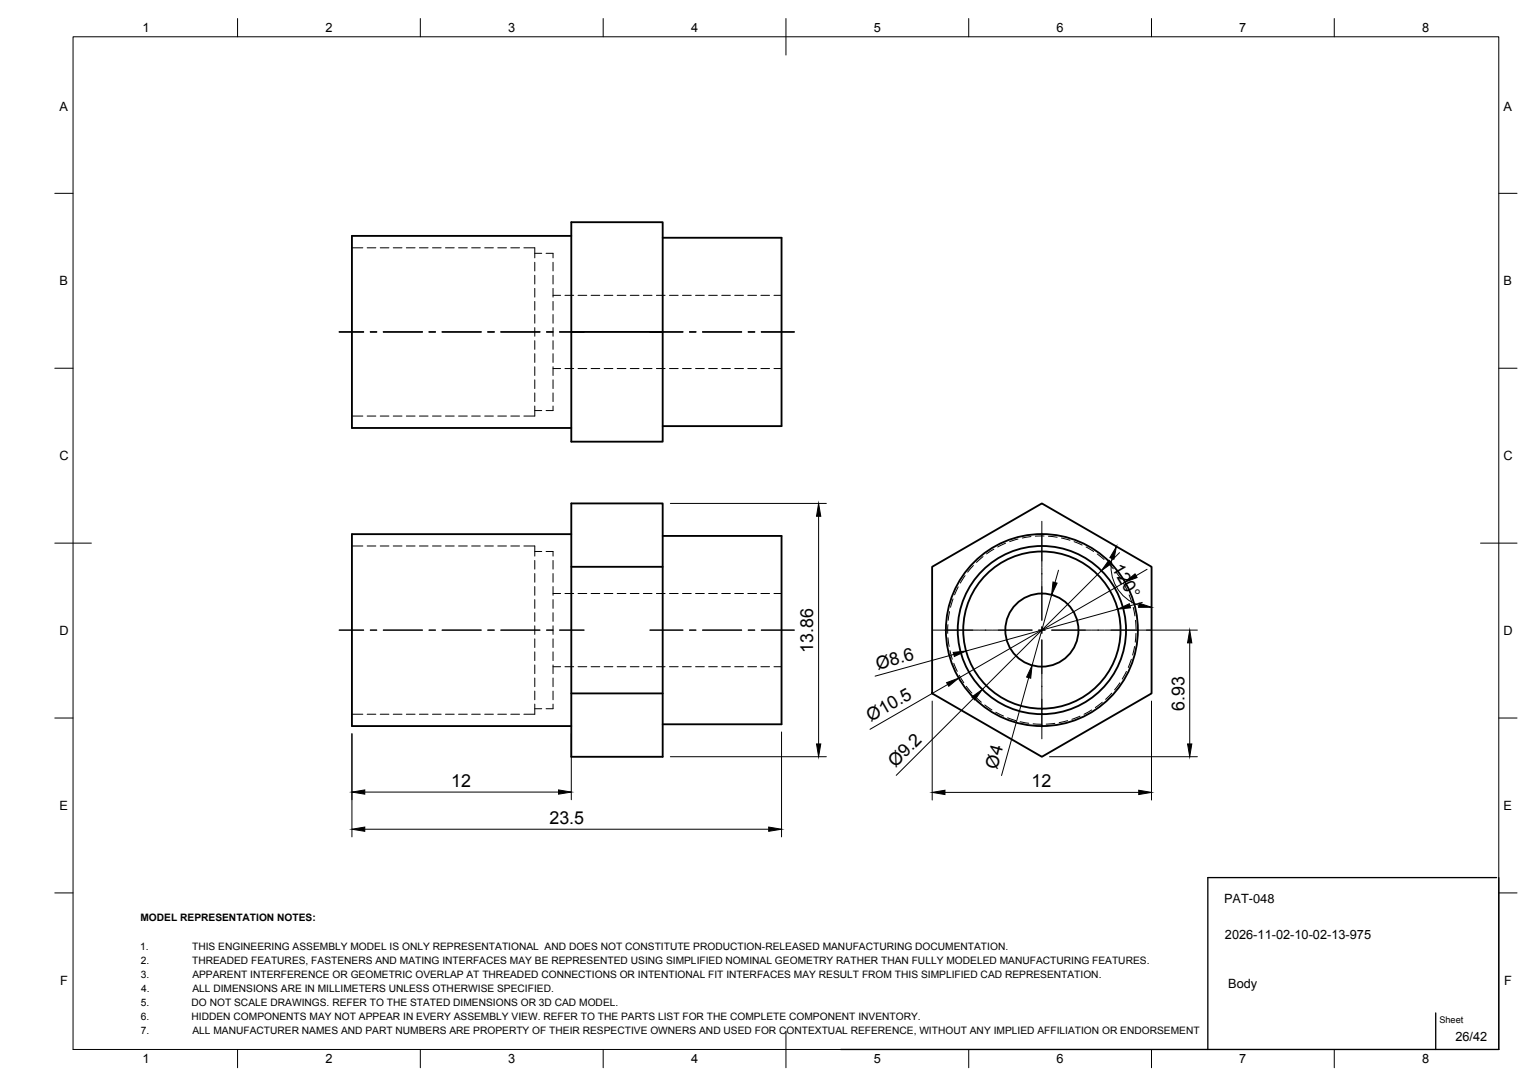
ISO-10303-21;
HEADER;
/* Generated by software containing ST-Developer
 * from STEP Tools, Inc. (www.steptools.com) 
 */

FILE_DESCRIPTION(
/* description */ ('Guided pneumatic stop gate'),
/* implementation_level */ '2;1');

FILE_NAME(
/* name */ 'Body.step',
/* time_stamp */ '2026-10-27T21:43:45-07:00',
/* author */ (''),
/* organization */ (''),
/* preprocessor_version */ 'ST-DEVELOPER v20.2',
/* originating_system */ 'Autodesk Translation Framework v15.17.0.0',
/* authorisation */ '');

FILE_SCHEMA (('AUTOMOTIVE_DESIGN { 1 0 10303 214 3 1 1 }'));
ENDSEC;

DATA;
#10=MECHANICAL_DESIGN_GEOMETRIC_PRESENTATION_REPRESENTATION('',(#546),#14392);
#462=SHAPE_REPRESENTATION_RELATIONSHIP('SRR','None',#14597,#504);
#504=ADVANCED_BREP_SHAPE_REPRESENTATION('',(#587),#14359);
#546=STYLED_ITEM('',(#14870),#587);
#587=MANIFOLD_SOLID_BREP('Body1',#7887);
#682=FACE_BOUND('',#1842,.T.);
#683=FACE_BOUND('',#1844,.T.);
#684=FACE_BOUND('',#1846,.T.);
#685=FACE_BOUND('',#1854,.T.);
#686=FACE_BOUND('',#1857,.T.);
#687=FACE_BOUND('',#1861,.T.);
#948=PLANE('',#8728);
#949=PLANE('',#8730);
#950=PLANE('',#8732);
#951=PLANE('',#8734);
#952=PLANE('',#8735);
#953=PLANE('',#8736);
#954=PLANE('',#8737);
#955=PLANE('',#8738);
#956=PLANE('',#8739);
#957=PLANE('',#8740);
#958=PLANE('',#8744);
#959=PLANE('',#8749);
#1298=FACE_OUTER_BOUND('',#1840,.T.);
#1299=FACE_OUTER_BOUND('',#1841,.T.);
#1300=FACE_OUTER_BOUND('',#1843,.T.);
#1301=FACE_OUTER_BOUND('',#1845,.T.);
#1302=FACE_OUTER_BOUND('',#1847,.T.);
#1303=FACE_OUTER_BOUND('',#1848,.T.);
#1304=FACE_OUTER_BOUND('',#1849,.T.);
#1305=FACE_OUTER_BOUND('',#1850,.T.);
#1306=FACE_OUTER_BOUND('',#1851,.T.);
#1307=FACE_OUTER_BOUND('',#1852,.T.);
#1308=FACE_OUTER_BOUND('',#1853,.T.);
#1309=FACE_OUTER_BOUND('',#1855,.T.);
#1310=FACE_OUTER_BOUND('',#1856,.T.);
#1311=FACE_OUTER_BOUND('',#1858,.T.);
#1312=FACE_OUTER_BOUND('',#1859,.T.);
#1313=FACE_OUTER_BOUND('',#1860,.T.);
#1314=FACE_OUTER_BOUND('',#1862,.T.);
#1840=EDGE_LOOP('',(#6034,#6035,#6036,#6037));
#1841=EDGE_LOOP('',(#6038));
#1842=EDGE_LOOP('',(#6039));
#1843=EDGE_LOOP('',(#6040,#6041,#6042,#6043,#6044,#6045));
#1844=EDGE_LOOP('',(#6046));
#1845=EDGE_LOOP('',(#6047,#6048,#6049,#6050,#6051,#6052));
#1846=EDGE_LOOP('',(#6053));
#1847=EDGE_LOOP('',(#6054,#6055,#6056,#6057));
#1848=EDGE_LOOP('',(#6058,#6059,#6060,#6061));
#1849=EDGE_LOOP('',(#6062,#6063,#6064,#6065));
#1850=EDGE_LOOP('',(#6066,#6067,#6068,#6069));
#1851=EDGE_LOOP('',(#6070,#6071,#6072,#6073));
#1852=EDGE_LOOP('',(#6074,#6075,#6076,#6077));
#1853=EDGE_LOOP('',(#6078));
#1854=EDGE_LOOP('',(#6079));
#1855=EDGE_LOOP('',(#6080,#6081,#6082,#6083));
#1856=EDGE_LOOP('',(#6084));
#1857=EDGE_LOOP('',(#6085));
#1858=EDGE_LOOP('',(#6086,#6087,#6088,#6089));
#1859=EDGE_LOOP('',(#6090,#6091,#6092,#6093));
#1860=EDGE_LOOP('',(#6094));
#1861=EDGE_LOOP('',(#6095));
#1862=EDGE_LOOP('',(#6096,#6097,#6098,#6099));
#2491=LINE('',#12704,#3036);
#2492=LINE('',#12712,#3037);
#2493=LINE('',#12714,#3038);
#2494=LINE('',#12716,#3039);
#2495=LINE('',#12718,#3040);
#2496=LINE('',#12720,#3041);
#2497=LINE('',#12721,#3042);
#2498=LINE('',#12727,#3043);
#2499=LINE('',#12729,#3044);
#2500=LINE('',#12731,#3045);
#2501=LINE('',#12733,#3046);
#2502=LINE('',#12735,#3047);
#2503=LINE('',#12736,#3048);
#2504=LINE('',#12740,#3049);
#2505=LINE('',#12741,#3050);
#2506=LINE('',#12743,#3051);
#2507=LINE('',#12745,#3052);
#2508=LINE('',#12747,#3053);
#2509=LINE('',#12749,#3054);
#2510=LINE('',#12756,#3055);
#2511=LINE('',#12762,#3056);
#2512=LINE('',#12766,#3057);
#2513=LINE('',#12771,#3058);
#3036=VECTOR('',#10280,0.43);
#3037=VECTOR('',#10289,1.);
#3038=VECTOR('',#10290,1.);
#3039=VECTOR('',#10291,1.);
#3040=VECTOR('',#10292,1.);
#3041=VECTOR('',#10293,1.);
#3042=VECTOR('',#10294,1.);
#3043=VECTOR('',#10299,1.);
#3044=VECTOR('',#10300,1.);
#3045=VECTOR('',#10301,1.);
#3046=VECTOR('',#10302,1.);
#3047=VECTOR('',#10303,1.);
#3048=VECTOR('',#10304,1.);
#3049=VECTOR('',#10309,1.);
#3050=VECTOR('',#10310,1.);
#3051=VECTOR('',#10313,1.);
#3052=VECTOR('',#10316,1.);
#3053=VECTOR('',#10319,1.);
#3054=VECTOR('',#10322,1.);
#3055=VECTOR('',#10331,0.46);
#3056=VECTOR('',#10340,0.525);
#3057=VECTOR('',#10345,0.515);
#3058=VECTOR('',#10352,0.2);
#3500=CIRCLE('',#8726,0.43);
#3501=CIRCLE('',#8727,0.43);
#3502=CIRCLE('',#8729,0.2);
#3503=CIRCLE('',#8731,0.525);
#3504=CIRCLE('',#8733,0.515);
#3505=CIRCLE('',#8741,0.46);
#3506=CIRCLE('',#8743,0.46);
#3507=CIRCLE('',#8745,0.525);
#3508=CIRCLE('',#8748,0.515);
#3509=CIRCLE('',#8750,0.2);
#3963=VERTEX_POINT('',#12701);
#3964=VERTEX_POINT('',#12703);
#3965=VERTEX_POINT('',#12707);
#3966=VERTEX_POINT('',#12710);
#3967=VERTEX_POINT('',#12711);
#3968=VERTEX_POINT('',#12713);
#3969=VERTEX_POINT('',#12715);
#3970=VERTEX_POINT('',#12717);
#3971=VERTEX_POINT('',#12719);
#3972=VERTEX_POINT('',#12722);
#3973=VERTEX_POINT('',#12725);
#3974=VERTEX_POINT('',#12726);
#3975=VERTEX_POINT('',#12728);
#3976=VERTEX_POINT('',#12730);
#3977=VERTEX_POINT('',#12732);
#3978=VERTEX_POINT('',#12734);
#3979=VERTEX_POINT('',#12737);
#3980=VERTEX_POINT('',#12752);
#3981=VERTEX_POINT('',#12755);
#3982=VERTEX_POINT('',#12759);
#3983=VERTEX_POINT('',#12764);
#3984=VERTEX_POINT('',#12768);
#4715=EDGE_CURVE('',#3963,#3963,#3500,.T.);
#4716=EDGE_CURVE('',#3963,#3964,#2491,.T.);
#4717=EDGE_CURVE('',#3964,#3964,#3501,.T.);
#4718=EDGE_CURVE('',#3965,#3965,#3502,.T.);
#4719=EDGE_CURVE('',#3966,#3967,#2492,.T.);
#4720=EDGE_CURVE('',#3967,#3968,#2493,.T.);
#4721=EDGE_CURVE('',#3968,#3969,#2494,.T.);
#4722=EDGE_CURVE('',#3969,#3970,#2495,.T.);
#4723=EDGE_CURVE('',#3970,#3971,#2496,.T.);
#4724=EDGE_CURVE('',#3971,#3966,#2497,.T.);
#4725=EDGE_CURVE('',#3972,#3972,#3503,.T.);
#4726=EDGE_CURVE('',#3973,#3974,#2498,.T.);
#4727=EDGE_CURVE('',#3975,#3973,#2499,.T.);
#4728=EDGE_CURVE('',#3976,#3975,#2500,.T.);
#4729=EDGE_CURVE('',#3977,#3976,#2501,.T.);
#4730=EDGE_CURVE('',#3978,#3977,#2502,.T.);
#4731=EDGE_CURVE('',#3974,#3978,#2503,.T.);
#4732=EDGE_CURVE('',#3979,#3979,#3504,.T.);
#4733=EDGE_CURVE('',#3973,#3966,#2504,.T.);
#4734=EDGE_CURVE('',#3975,#3971,#2505,.T.);
#4735=EDGE_CURVE('',#3976,#3970,#2506,.T.);
#4736=EDGE_CURVE('',#3977,#3969,#2507,.T.);
#4737=EDGE_CURVE('',#3978,#3968,#2508,.T.);
#4738=EDGE_CURVE('',#3974,#3967,#2509,.T.);
#4739=EDGE_CURVE('',#3980,#3980,#3505,.T.);
#4740=EDGE_CURVE('',#3980,#3981,#2510,.T.);
#4741=EDGE_CURVE('',#3981,#3981,#3506,.T.);
#4742=EDGE_CURVE('',#3982,#3982,#3507,.T.);
#4743=EDGE_CURVE('',#3972,#3982,#2511,.T.);
#4744=EDGE_CURVE('',#3983,#3983,#3508,.T.);
#4745=EDGE_CURVE('',#3983,#3979,#2512,.T.);
#4746=EDGE_CURVE('',#3984,#3984,#3509,.T.);
#4747=EDGE_CURVE('',#3984,#3965,#2513,.T.);
#6034=ORIENTED_EDGE('',*,*,#4715,.F.);
#6035=ORIENTED_EDGE('',*,*,#4716,.T.);
#6036=ORIENTED_EDGE('',*,*,#4717,.F.);
#6037=ORIENTED_EDGE('',*,*,#4716,.F.);
#6038=ORIENTED_EDGE('',*,*,#4715,.T.);
#6039=ORIENTED_EDGE('',*,*,#4718,.F.);
#6040=ORIENTED_EDGE('',*,*,#4719,.T.);
#6041=ORIENTED_EDGE('',*,*,#4720,.T.);
#6042=ORIENTED_EDGE('',*,*,#4721,.T.);
#6043=ORIENTED_EDGE('',*,*,#4722,.T.);
#6044=ORIENTED_EDGE('',*,*,#4723,.T.);
#6045=ORIENTED_EDGE('',*,*,#4724,.T.);
#6046=ORIENTED_EDGE('',*,*,#4725,.T.);
#6047=ORIENTED_EDGE('',*,*,#4726,.F.);
#6048=ORIENTED_EDGE('',*,*,#4727,.F.);
#6049=ORIENTED_EDGE('',*,*,#4728,.F.);
#6050=ORIENTED_EDGE('',*,*,#4729,.F.);
#6051=ORIENTED_EDGE('',*,*,#4730,.F.);
#6052=ORIENTED_EDGE('',*,*,#4731,.F.);
#6053=ORIENTED_EDGE('',*,*,#4732,.F.);
#6054=ORIENTED_EDGE('',*,*,#4727,.T.);
#6055=ORIENTED_EDGE('',*,*,#4733,.T.);
#6056=ORIENTED_EDGE('',*,*,#4724,.F.);
#6057=ORIENTED_EDGE('',*,*,#4734,.F.);
#6058=ORIENTED_EDGE('',*,*,#4728,.T.);
#6059=ORIENTED_EDGE('',*,*,#4734,.T.);
#6060=ORIENTED_EDGE('',*,*,#4723,.F.);
#6061=ORIENTED_EDGE('',*,*,#4735,.F.);
#6062=ORIENTED_EDGE('',*,*,#4729,.T.);
#6063=ORIENTED_EDGE('',*,*,#4735,.T.);
#6064=ORIENTED_EDGE('',*,*,#4722,.F.);
#6065=ORIENTED_EDGE('',*,*,#4736,.F.);
#6066=ORIENTED_EDGE('',*,*,#4730,.T.);
#6067=ORIENTED_EDGE('',*,*,#4736,.T.);
#6068=ORIENTED_EDGE('',*,*,#4721,.F.);
#6069=ORIENTED_EDGE('',*,*,#4737,.F.);
#6070=ORIENTED_EDGE('',*,*,#4731,.T.);
#6071=ORIENTED_EDGE('',*,*,#4737,.T.);
#6072=ORIENTED_EDGE('',*,*,#4720,.F.);
#6073=ORIENTED_EDGE('',*,*,#4738,.F.);
#6074=ORIENTED_EDGE('',*,*,#4726,.T.);
#6075=ORIENTED_EDGE('',*,*,#4738,.T.);
#6076=ORIENTED_EDGE('',*,*,#4719,.F.);
#6077=ORIENTED_EDGE('',*,*,#4733,.F.);
#6078=ORIENTED_EDGE('',*,*,#4739,.F.);
#6079=ORIENTED_EDGE('',*,*,#4717,.T.);
#6080=ORIENTED_EDGE('',*,*,#4739,.T.);
#6081=ORIENTED_EDGE('',*,*,#4740,.T.);
#6082=ORIENTED_EDGE('',*,*,#4741,.F.);
#6083=ORIENTED_EDGE('',*,*,#4740,.F.);
#6084=ORIENTED_EDGE('',*,*,#4742,.F.);
#6085=ORIENTED_EDGE('',*,*,#4741,.T.);
#6086=ORIENTED_EDGE('',*,*,#4725,.F.);
#6087=ORIENTED_EDGE('',*,*,#4743,.T.);
#6088=ORIENTED_EDGE('',*,*,#4742,.T.);
#6089=ORIENTED_EDGE('',*,*,#4743,.F.);
#6090=ORIENTED_EDGE('',*,*,#4744,.F.);
#6091=ORIENTED_EDGE('',*,*,#4745,.T.);
#6092=ORIENTED_EDGE('',*,*,#4732,.T.);
#6093=ORIENTED_EDGE('',*,*,#4745,.F.);
#6094=ORIENTED_EDGE('',*,*,#4744,.T.);
#6095=ORIENTED_EDGE('',*,*,#4746,.F.);
#6096=ORIENTED_EDGE('',*,*,#4746,.T.);
#6097=ORIENTED_EDGE('',*,*,#4747,.T.);
#6098=ORIENTED_EDGE('',*,*,#4718,.T.);
#6099=ORIENTED_EDGE('',*,*,#4747,.F.);
#7299=CYLINDRICAL_SURFACE('',#8725,0.43);
#7300=CYLINDRICAL_SURFACE('',#8742,0.46);
#7301=CYLINDRICAL_SURFACE('',#8746,0.525);
#7302=CYLINDRICAL_SURFACE('',#8747,0.515);
#7303=CYLINDRICAL_SURFACE('',#8751,0.2);
#7580=ADVANCED_FACE('',(#1298),#7299,.F.);
#7581=ADVANCED_FACE('',(#1299,#682),#948,.T.);
#7582=ADVANCED_FACE('',(#1300,#683),#949,.T.);
#7583=ADVANCED_FACE('',(#1301,#684),#950,.F.);
#7584=ADVANCED_FACE('',(#1302),#951,.T.);
#7585=ADVANCED_FACE('',(#1303),#952,.T.);
#7586=ADVANCED_FACE('',(#1304),#953,.T.);
#7587=ADVANCED_FACE('',(#1305),#954,.T.);
#7588=ADVANCED_FACE('',(#1306),#955,.T.);
#7589=ADVANCED_FACE('',(#1307),#956,.T.);
#7590=ADVANCED_FACE('',(#1308,#685),#957,.T.);
#7591=ADVANCED_FACE('',(#1309),#7300,.F.);
#7592=ADVANCED_FACE('',(#1310,#686),#958,.T.);
#7593=ADVANCED_FACE('',(#1311),#7301,.T.);
#7594=ADVANCED_FACE('',(#1312),#7302,.T.);
#7595=ADVANCED_FACE('',(#1313,#687),#959,.T.);
#7596=ADVANCED_FACE('',(#1314),#7303,.F.);
#7887=CLOSED_SHELL('',(#7580,#7581,#7582,#7583,#7584,#7585,#7586,#7587,
#7588,#7589,#7590,#7591,#7592,#7593,#7594,#7595,#7596));
#8724=AXIS2_PLACEMENT_3D('',#12699,#10274,#10275);
#8725=AXIS2_PLACEMENT_3D('',#12700,#10276,#10277);
#8726=AXIS2_PLACEMENT_3D('',#12702,#10278,#10279);
#8727=AXIS2_PLACEMENT_3D('',#12705,#10281,#10282);
#8728=AXIS2_PLACEMENT_3D('',#12706,#10283,#10284);
#8729=AXIS2_PLACEMENT_3D('',#12708,#10285,#10286);
#8730=AXIS2_PLACEMENT_3D('',#12709,#10287,#10288);
#8731=AXIS2_PLACEMENT_3D('',#12723,#10295,#10296);
#8732=AXIS2_PLACEMENT_3D('',#12724,#10297,#10298);
#8733=AXIS2_PLACEMENT_3D('',#12738,#10305,#10306);
#8734=AXIS2_PLACEMENT_3D('',#12739,#10307,#10308);
#8735=AXIS2_PLACEMENT_3D('',#12742,#10311,#10312);
#8736=AXIS2_PLACEMENT_3D('',#12744,#10314,#10315);
#8737=AXIS2_PLACEMENT_3D('',#12746,#10317,#10318);
#8738=AXIS2_PLACEMENT_3D('',#12748,#10320,#10321);
#8739=AXIS2_PLACEMENT_3D('',#12750,#10323,#10324);
#8740=AXIS2_PLACEMENT_3D('',#12751,#10325,#10326);
#8741=AXIS2_PLACEMENT_3D('',#12753,#10327,#10328);
#8742=AXIS2_PLACEMENT_3D('',#12754,#10329,#10330);
#8743=AXIS2_PLACEMENT_3D('',#12757,#10332,#10333);
#8744=AXIS2_PLACEMENT_3D('',#12758,#10334,#10335);
#8745=AXIS2_PLACEMENT_3D('',#12760,#10336,#10337);
#8746=AXIS2_PLACEMENT_3D('',#12761,#10338,#10339);
#8747=AXIS2_PLACEMENT_3D('',#12763,#10341,#10342);
#8748=AXIS2_PLACEMENT_3D('',#12765,#10343,#10344);
#8749=AXIS2_PLACEMENT_3D('',#12767,#10346,#10347);
#8750=AXIS2_PLACEMENT_3D('',#12769,#10348,#10349);
#8751=AXIS2_PLACEMENT_3D('',#12770,#10350,#10351);
#10274=DIRECTION('axis',(0.,0.,1.));
#10275=DIRECTION('refdir',(1.,0.,0.));
#10276=DIRECTION('center_axis',(0.,1.,0.));
#10277=DIRECTION('ref_axis',(1.,0.,0.));
#10278=DIRECTION('center_axis',(0.,1.,0.));
#10279=DIRECTION('ref_axis',(1.,0.,0.));
#10280=DIRECTION('',(0.,1.,0.));
#10281=DIRECTION('center_axis',(0.,-1.,0.));
#10282=DIRECTION('ref_axis',(1.,0.,0.));
#10283=DIRECTION('center_axis',(0.,1.,0.));
#10284=DIRECTION('ref_axis',(1.,0.,0.));
#10285=DIRECTION('center_axis',(0.,1.,0.));
#10286=DIRECTION('ref_axis',(1.,0.,0.));
#10287=DIRECTION('center_axis',(0.,1.,0.));
#10288=DIRECTION('ref_axis',(1.,0.,0.));
#10289=DIRECTION('',(0.5,0.,-0.866025403784439));
#10290=DIRECTION('',(-0.5,0.,-0.866025403784439));
#10291=DIRECTION('',(-1.,0.,-1.60246890531964E-16));
#10292=DIRECTION('',(-0.5,0.,0.866025403784439));
#10293=DIRECTION('',(0.5,0.,0.866025403784439));
#10294=DIRECTION('',(1.,0.,1.60246890531964E-16));
#10295=DIRECTION('center_axis',(0.,-1.,0.));
#10296=DIRECTION('ref_axis',(1.,0.,0.));
#10297=DIRECTION('center_axis',(0.,1.,0.));
#10298=DIRECTION('ref_axis',(1.,0.,0.));
#10299=DIRECTION('',(0.5,0.,-0.866025403784439));
#10300=DIRECTION('',(1.,0.,1.60246890531964E-16));
#10301=DIRECTION('',(0.5,0.,0.866025403784439));
#10302=DIRECTION('',(-0.5,0.,0.866025403784439));
#10303=DIRECTION('',(-1.,0.,-1.60246890531964E-16));
#10304=DIRECTION('',(-0.5,0.,-0.866025403784439));
#10305=DIRECTION('center_axis',(0.,-1.,0.));
#10306=DIRECTION('ref_axis',(1.,0.,0.));
#10307=DIRECTION('center_axis',(-1.60246890531964E-16,0.,1.));
#10308=DIRECTION('ref_axis',(1.,0.,1.60246890531964E-16));
#10309=DIRECTION('',(0.,1.,0.));
#10310=DIRECTION('',(0.,1.,0.));
#10311=DIRECTION('center_axis',(-0.866025403784439,0.,0.5));
#10312=DIRECTION('ref_axis',(0.5,0.,0.866025403784439));
#10313=DIRECTION('',(0.,1.,0.));
#10314=DIRECTION('center_axis',(-0.866025403784439,0.,-0.5));
#10315=DIRECTION('ref_axis',(-0.5,0.,0.866025403784439));
#10316=DIRECTION('',(0.,1.,0.));
#10317=DIRECTION('center_axis',(1.60246890531964E-16,0.,-1.));
#10318=DIRECTION('ref_axis',(-1.,0.,-1.60246890531964E-16));
#10319=DIRECTION('',(0.,1.,0.));
#10320=DIRECTION('center_axis',(0.866025403784439,0.,-0.5));
#10321=DIRECTION('ref_axis',(-0.5,0.,-0.866025403784439));
#10322=DIRECTION('',(0.,1.,0.));
#10323=DIRECTION('center_axis',(0.866025403784439,0.,0.5));
#10324=DIRECTION('ref_axis',(0.5,0.,-0.866025403784439));
#10325=DIRECTION('center_axis',(0.,1.,0.));
#10326=DIRECTION('ref_axis',(0.,0.,1.));
#10327=DIRECTION('center_axis',(0.,-1.,0.));
#10328=DIRECTION('ref_axis',(1.,0.,0.));
#10329=DIRECTION('center_axis',(0.,-1.,0.));
#10330=DIRECTION('ref_axis',(1.,0.,0.));
#10331=DIRECTION('',(0.,1.,0.));
#10332=DIRECTION('center_axis',(0.,-1.,0.));
#10333=DIRECTION('ref_axis',(1.,0.,0.));
#10334=DIRECTION('center_axis',(0.,1.,0.));
#10335=DIRECTION('ref_axis',(0.,0.,1.));
#10336=DIRECTION('center_axis',(0.,-1.,0.));
#10337=DIRECTION('ref_axis',(1.,0.,0.));
#10338=DIRECTION('center_axis',(0.,-1.,0.));
#10339=DIRECTION('ref_axis',(1.,0.,0.));
#10340=DIRECTION('',(0.,1.,0.));
#10341=DIRECTION('center_axis',(0.,-1.,0.));
#10342=DIRECTION('ref_axis',(1.,0.,0.));
#10343=DIRECTION('center_axis',(0.,-1.,0.));
#10344=DIRECTION('ref_axis',(1.,0.,0.));
#10345=DIRECTION('',(0.,1.,0.));
#10346=DIRECTION('center_axis',(0.,-1.,0.));
#10347=DIRECTION('ref_axis',(0.,0.,-1.));
#10348=DIRECTION('center_axis',(0.,-1.,0.));
#10349=DIRECTION('ref_axis',(1.,0.,0.));
#10350=DIRECTION('center_axis',(0.,-1.,0.));
#10351=DIRECTION('ref_axis',(1.,0.,0.));
#10352=DIRECTION('',(0.,1.,0.));
#12699=CARTESIAN_POINT('',(0.,0.,0.));
#12700=CARTESIAN_POINT('Origin',(0.,0.6,0.));
#12701=CARTESIAN_POINT('',(-0.43,0.6,5.26598123633362E-17));
#12702=CARTESIAN_POINT('Origin',(0.,0.6,0.));
#12703=CARTESIAN_POINT('',(-0.43,0.7,-5.26598123633362E-17));
#12704=CARTESIAN_POINT('',(-0.43,0.6,5.26598123633362E-17));
#12705=CARTESIAN_POINT('Origin',(0.,0.7,0.));
#12706=CARTESIAN_POINT('Origin',(0.,0.6,0.));
#12707=CARTESIAN_POINT('',(-0.2,0.6,2.44929359829471E-17));
#12708=CARTESIAN_POINT('Origin',(0.,0.6,0.));
#12709=CARTESIAN_POINT('Origin',(0.,0.5,-1.11022302462516E-16));
#12710=CARTESIAN_POINT('',(0.346410161513776,0.5,0.6));
#12711=CARTESIAN_POINT('',(0.692820323027551,0.5,0.));
#12712=CARTESIAN_POINT('',(0.346410161513776,0.5,0.6));
#12713=CARTESIAN_POINT('',(0.346410161513776,0.5,-0.6));
#12714=CARTESIAN_POINT('',(0.692820323027551,0.5,0.));
#12715=CARTESIAN_POINT('',(-0.346410161513775,0.5,-0.6));
#12716=CARTESIAN_POINT('',(0.346410161513776,0.5,-0.6));
#12717=CARTESIAN_POINT('',(-0.692820323027551,0.5,-8.48460190979926E-17));
#12718=CARTESIAN_POINT('',(-0.346410161513775,0.5,-0.6));
#12719=CARTESIAN_POINT('',(-0.346410161513776,0.5,0.6));
#12720=CARTESIAN_POINT('',(-0.692820323027551,0.5,-8.48460190979926E-17));
#12721=CARTESIAN_POINT('',(-0.346410161513776,0.5,0.6));
#12722=CARTESIAN_POINT('',(-0.525,0.5,-6.4293956955236E-17));
#12723=CARTESIAN_POINT('Origin',(0.,0.5,0.));
#12724=CARTESIAN_POINT('Origin',(0.,0.,-1.11022302462516E-16));
#12725=CARTESIAN_POINT('',(0.346410161513776,0.,0.6));
#12726=CARTESIAN_POINT('',(0.692820323027551,0.,0.));
#12727=CARTESIAN_POINT('',(0.346410161513776,0.,0.6));
#12728=CARTESIAN_POINT('',(-0.346410161513776,0.,0.6));
#12729=CARTESIAN_POINT('',(-0.346410161513776,0.,0.6));
#12730=CARTESIAN_POINT('',(-0.692820323027551,0.,-8.48460190979926E-17));
#12731=CARTESIAN_POINT('',(-0.692820323027551,0.,-8.48460190979926E-17));
#12732=CARTESIAN_POINT('',(-0.346410161513775,0.,-0.6));
#12733=CARTESIAN_POINT('',(-0.346410161513775,0.,-0.6));
#12734=CARTESIAN_POINT('',(0.346410161513776,0.,-0.6));
#12735=CARTESIAN_POINT('',(0.346410161513776,0.,-0.6));
#12736=CARTESIAN_POINT('',(0.692820323027551,0.,0.));
#12737=CARTESIAN_POINT('',(-0.515,0.,-6.30693101560887E-17));
#12738=CARTESIAN_POINT('Origin',(0.,0.,0.));
#12739=CARTESIAN_POINT('Origin',(-0.346410161513776,0.,0.6));
#12740=CARTESIAN_POINT('',(0.346410161513776,0.,0.6));
#12741=CARTESIAN_POINT('',(-0.346410161513776,0.,0.6));
#12742=CARTESIAN_POINT('Origin',(-0.692820323027551,0.,-8.48460190979926E-17));
#12743=CARTESIAN_POINT('',(-0.692820323027551,0.,-8.48460190979926E-17));
#12744=CARTESIAN_POINT('Origin',(-0.346410161513775,0.,-0.6));
#12745=CARTESIAN_POINT('',(-0.346410161513775,0.,-0.6));
#12746=CARTESIAN_POINT('Origin',(0.346410161513776,0.,-0.6));
#12747=CARTESIAN_POINT('',(0.346410161513776,0.,-0.6));
#12748=CARTESIAN_POINT('Origin',(0.692820323027551,0.,0.));
#12749=CARTESIAN_POINT('',(0.692820323027551,0.,0.));
#12750=CARTESIAN_POINT('Origin',(0.346410161513776,0.,0.6));
#12751=CARTESIAN_POINT('Origin',(0.46,0.7,0.));
#12752=CARTESIAN_POINT('',(-0.46,0.7,-5.63337527607782E-17));
#12753=CARTESIAN_POINT('Origin',(0.,0.7,0.));
#12754=CARTESIAN_POINT('Origin',(0.,1.2,0.));
#12755=CARTESIAN_POINT('',(-0.46,1.7,-5.63337527607782E-17));
#12756=CARTESIAN_POINT('',(-0.46,1.2,-5.63337527607782E-17));
#12757=CARTESIAN_POINT('Origin',(0.,1.7,0.));
#12758=CARTESIAN_POINT('Origin',(0.525,1.7,0.));
#12759=CARTESIAN_POINT('',(-0.525,1.7,-6.4293956955236E-17));
#12760=CARTESIAN_POINT('Origin',(0.,1.7,0.));
#12761=CARTESIAN_POINT('Origin',(0.,1.1,0.));
#12762=CARTESIAN_POINT('',(-0.525,1.1,-6.4293956955236E-17));
#12763=CARTESIAN_POINT('Origin',(0.,-0.325,0.));
#12764=CARTESIAN_POINT('',(-0.515,-0.65,-6.30693101560887E-17));
#12765=CARTESIAN_POINT('Origin',(0.,-0.65,0.));
#12766=CARTESIAN_POINT('',(-0.515,-0.325,-6.30693101560887E-17));
#12767=CARTESIAN_POINT('Origin',(0.2,-0.65,0.));
#12768=CARTESIAN_POINT('',(-0.2,-0.65,-2.44929359829471E-17));
#12769=CARTESIAN_POINT('Origin',(0.,-0.65,0.));
#12770=CARTESIAN_POINT('Origin',(0.,0.0249999999999999,0.));
#12771=CARTESIAN_POINT('',(-0.2,0.0249999999999999,-2.44929359829471E-17));
#14311=UNCERTAINTY_MEASURE_WITH_UNIT(LENGTH_MEASURE(0.001),#14393,
'DISTANCE_ACCURACY_VALUE',
'Maximum model space distance between geometric entities at asserted c
onnectivities');
#14344=UNCERTAINTY_MEASURE_WITH_UNIT(LENGTH_MEASURE(0.001),#14393,
'DISTANCE_ACCURACY_VALUE',
'Maximum model space distance between geometric entities at asserted c
onnectivities');
#14359=(
GEOMETRIC_REPRESENTATION_CONTEXT(3)
GLOBAL_UNCERTAINTY_ASSIGNED_CONTEXT((#14311))
GLOBAL_UNIT_ASSIGNED_CONTEXT((#14393,#14395,#14396))
REPRESENTATION_CONTEXT('','3D')
);
#14392=(
GEOMETRIC_REPRESENTATION_CONTEXT(3)
GLOBAL_UNCERTAINTY_ASSIGNED_CONTEXT((#14344))
GLOBAL_UNIT_ASSIGNED_CONTEXT((#14393,#14395,#14396))
REPRESENTATION_CONTEXT('','3D')
);
#14393=(
LENGTH_UNIT()
NAMED_UNIT(*)
SI_UNIT(.CENTI.,.METRE.)
);
#14395=(
NAMED_UNIT(*)
PLANE_ANGLE_UNIT()
SI_UNIT($,.RADIAN.)
);
#14396=(
NAMED_UNIT(*)
SI_UNIT($,.STERADIAN.)
SOLID_ANGLE_UNIT()
);
#14411=SHAPE_DEFINITION_REPRESENTATION(#14458,#14597);
#14458=PRODUCT_DEFINITION_SHAPE('',$,#14645);
#14597=SHAPE_REPRESENTATION('',(#8724),#14359);
#14630=PRODUCT_DEFINITION_CONTEXT('part definition',#14773,'design');
#14645=PRODUCT_DEFINITION('Body','Body',#14692,#14630);
#14692=PRODUCT_DEFINITION_FORMATION('',$,#14789);
#14773=APPLICATION_CONTEXT(
'Core Data for Automotive Mechanical Design Process');
#14774=PRODUCT_CONTEXT('part definition',#14773,'mechanical');
#14789=PRODUCT('Body','Body','Body',(#14774));
#14864=COLOUR_RGB('Dark Blue',0.08,0.2,0.34);
#14865=FILL_AREA_STYLE_COLOUR('',#14864);
#14866=FILL_AREA_STYLE('',(#14865));
#14867=SURFACE_STYLE_FILL_AREA(#14866);
#14868=SURFACE_SIDE_STYLE('',(#14867));
#14869=SURFACE_STYLE_USAGE(.BOTH.,#14868);
#14870=PRESENTATION_STYLE_ASSIGNMENT((#14869));
ENDSEC;
END-ISO-10303-21;
